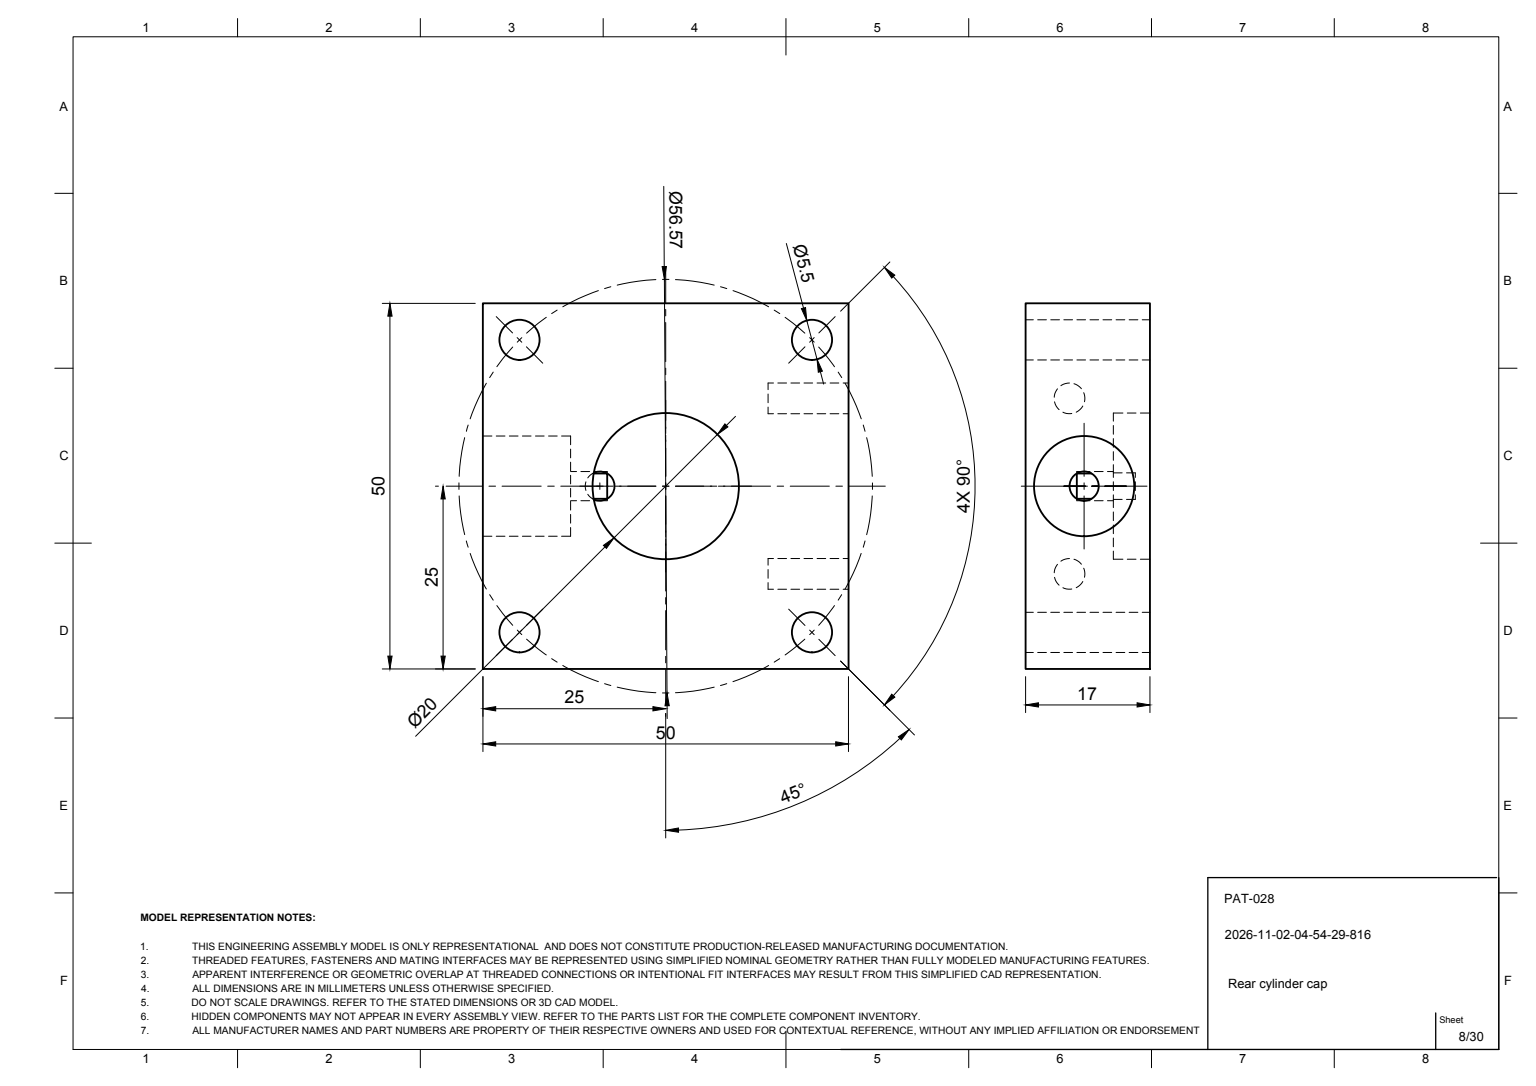
ISO-10303-21;
HEADER;
/* Generated by software containing ST-Developer
 * from STEP Tools, Inc. (www.steptools.com) 
 */

FILE_DESCRIPTION(
/* description */ ('Cylinder foot and clevis mount kit'),
/* implementation_level */ '2;1');

FILE_NAME(
/* name */ 'Rear cylinder cap.step',
/* time_stamp */ '2026-10-27T20:10:43-07:00',
/* author */ (''),
/* organization */ (''),
/* preprocessor_version */ 'ST-DEVELOPER v20.2',
/* originating_system */ 'Autodesk Translation Framework v15.17.0.0',
/* authorisation */ '');

FILE_SCHEMA (('AUTOMOTIVE_DESIGN { 1 0 10303 214 3 1 1 }'));
ENDSEC;

DATA;
#10=MECHANICAL_DESIGN_GEOMETRIC_PRESENTATION_REPRESENTATION('',(#341),#9102);
#285=SHAPE_REPRESENTATION_RELATIONSHIP('SRR','None',#9232,#313);
#313=ADVANCED_BREP_SHAPE_REPRESENTATION('',(#369),#9075);
#341=STYLED_ITEM('',(#9446),#369);
#369=MANIFOLD_SOLID_BREP('Body1',#4927);
#417=FACE_BOUND('',#1113,.T.);
#418=FACE_BOUND('',#1120,.T.);
#419=FACE_BOUND('',#1121,.T.);
#420=FACE_BOUND('',#1122,.T.);
#421=FACE_BOUND('',#1123,.T.);
#422=FACE_BOUND('',#1126,.T.);
#423=FACE_BOUND('',#1127,.T.);
#424=FACE_BOUND('',#1128,.T.);
#425=FACE_BOUND('',#1129,.T.);
#426=FACE_BOUND('',#1130,.T.);
#427=FACE_BOUND('',#1133,.T.);
#428=FACE_BOUND('',#1135,.T.);
#429=FACE_BOUND('',#1136,.T.);
#502=ELLIPSE('',#5409,0.282842712474618,0.2);
#503=ELLIPSE('',#5410,0.282842712474618,0.2);
#504=ELLIPSE('',#5411,0.282842712474618,0.2);
#505=ELLIPSE('',#5414,0.282842712474618,0.2);
#506=ELLIPSE('',#5415,0.282842712474618,0.2);
#507=ELLIPSE('',#5417,0.282842712474618,0.2);
#508=ELLIPSE('',#5418,0.282842712474618,0.2);
#550=PLANE('',#5395);
#551=PLANE('',#5399);
#552=PLANE('',#5400);
#553=PLANE('',#5402);
#554=PLANE('',#5404);
#555=PLANE('',#5419);
#556=PLANE('',#5421);
#557=PLANE('',#5423);
#558=PLANE('',#5425);
#559=PLANE('',#5431);
#560=PLANE('',#5437);
#561=PLANE('',#5452);
#562=PLANE('',#5453);
#563=PLANE('',#5454);
#564=PLANE('',#5455);
#565=PLANE('',#5456);
#566=PLANE('',#5457);
#762=FACE_OUTER_BOUND('',#1093,.T.);
#763=FACE_OUTER_BOUND('',#1094,.T.);
#764=FACE_OUTER_BOUND('',#1095,.T.);
#765=FACE_OUTER_BOUND('',#1096,.T.);
#766=FACE_OUTER_BOUND('',#1097,.T.);
#767=FACE_OUTER_BOUND('',#1098,.T.);
#768=FACE_OUTER_BOUND('',#1099,.T.);
#769=FACE_OUTER_BOUND('',#1100,.T.);
#770=FACE_OUTER_BOUND('',#1101,.T.);
#771=FACE_OUTER_BOUND('',#1102,.T.);
#772=FACE_OUTER_BOUND('',#1103,.T.);
#773=FACE_OUTER_BOUND('',#1104,.T.);
#774=FACE_OUTER_BOUND('',#1105,.T.);
#775=FACE_OUTER_BOUND('',#1106,.T.);
#776=FACE_OUTER_BOUND('',#1107,.T.);
#777=FACE_OUTER_BOUND('',#1108,.T.);
#778=FACE_OUTER_BOUND('',#1109,.T.);
#779=FACE_OUTER_BOUND('',#1110,.T.);
#780=FACE_OUTER_BOUND('',#1111,.T.);
#781=FACE_OUTER_BOUND('',#1112,.T.);
#782=FACE_OUTER_BOUND('',#1114,.T.);
#783=FACE_OUTER_BOUND('',#1115,.T.);
#784=FACE_OUTER_BOUND('',#1116,.T.);
#785=FACE_OUTER_BOUND('',#1117,.T.);
#786=FACE_OUTER_BOUND('',#1118,.T.);
#787=FACE_OUTER_BOUND('',#1119,.T.);
#788=FACE_OUTER_BOUND('',#1124,.T.);
#789=FACE_OUTER_BOUND('',#1125,.T.);
#790=FACE_OUTER_BOUND('',#1131,.T.);
#791=FACE_OUTER_BOUND('',#1132,.T.);
#792=FACE_OUTER_BOUND('',#1134,.T.);
#1093=EDGE_LOOP('',(#3591,#3592,#3593,#3594));
#1094=EDGE_LOOP('',(#3595));
#1095=EDGE_LOOP('',(#3596,#3597,#3598,#3599));
#1096=EDGE_LOOP('',(#3600));
#1097=EDGE_LOOP('',(#3601,#3602));
#1098=EDGE_LOOP('',(#3603,#3604));
#1099=EDGE_LOOP('',(#3605,#3606));
#1100=EDGE_LOOP('',(#3607,#3608,#3609,#3610,#3611,#3612,#3613,#3614,#3615,
#3616,#3617,#3618,#3619));
#1101=EDGE_LOOP('',(#3620,#3621,#3622));
#1102=EDGE_LOOP('',(#3623,#3624,#3625));
#1103=EDGE_LOOP('',(#3626,#3627));
#1104=EDGE_LOOP('',(#3628,#3629));
#1105=EDGE_LOOP('',(#3630,#3631));
#1106=EDGE_LOOP('',(#3632,#3633));
#1107=EDGE_LOOP('',(#3634,#3635,#3636));
#1108=EDGE_LOOP('',(#3637,#3638,#3639));
#1109=EDGE_LOOP('',(#3640,#3641,#3642,#3643,#3644,#3645,#3646,#3647,#3648));
#1110=EDGE_LOOP('',(#3649,#3650,#3651,#3652));
#1111=EDGE_LOOP('',(#3653,#3654,#3655,#3656));
#1112=EDGE_LOOP('',(#3657));
#1113=EDGE_LOOP('',(#3658));
#1114=EDGE_LOOP('',(#3659,#3660,#3661,#3662));
#1115=EDGE_LOOP('',(#3663,#3664,#3665,#3666));
#1116=EDGE_LOOP('',(#3667,#3668,#3669,#3670));
#1117=EDGE_LOOP('',(#3671,#3672,#3673,#3674));
#1118=EDGE_LOOP('',(#3675,#3676,#3677,#3678,#3679,#3680,#3681,#3682));
#1119=EDGE_LOOP('',(#3683,#3684,#3685,#3686));
#1120=EDGE_LOOP('',(#3687));
#1121=EDGE_LOOP('',(#3688));
#1122=EDGE_LOOP('',(#3689));
#1123=EDGE_LOOP('',(#3690));
#1124=EDGE_LOOP('',(#3691,#3692,#3693,#3694));
#1125=EDGE_LOOP('',(#3695,#3696,#3697,#3698));
#1126=EDGE_LOOP('',(#3699));
#1127=EDGE_LOOP('',(#3700));
#1128=EDGE_LOOP('',(#3701));
#1129=EDGE_LOOP('',(#3702));
#1130=EDGE_LOOP('',(#3703));
#1131=EDGE_LOOP('',(#3704,#3705,#3706,#3707));
#1132=EDGE_LOOP('',(#3708,#3709,#3710,#3711));
#1133=EDGE_LOOP('',(#3712));
#1134=EDGE_LOOP('',(#3713,#3714,#3715,#3716));
#1135=EDGE_LOOP('',(#3717));
#1136=EDGE_LOOP('',(#3718));
#1492=LINE('',#7797,#1841);
#1493=LINE('',#7804,#1842);
#1494=LINE('',#7810,#1843);
#1495=LINE('',#7814,#1844);
#1496=LINE('',#7818,#1845);
#1497=LINE('',#7823,#1846);
#1498=LINE('',#7827,#1847);
#1499=LINE('',#7831,#1848);
#1500=LINE('',#7836,#1849);
#1501=LINE('',#7838,#1850);
#1502=LINE('',#7859,#1851);
#1503=LINE('',#7869,#1852);
#1504=LINE('',#7876,#1853);
#1505=LINE('',#7882,#1854);
#1506=LINE('',#7888,#1855);
#1507=LINE('',#7894,#1856);
#1508=LINE('',#7899,#1857);
#1509=LINE('',#7903,#1858);
#1510=LINE('',#7905,#1859);
#1511=LINE('',#7907,#1860);
#1512=LINE('',#7908,#1861);
#1513=LINE('',#7911,#1862);
#1514=LINE('',#7913,#1863);
#1515=LINE('',#7914,#1864);
#1516=LINE('',#7917,#1865);
#1517=LINE('',#7919,#1866);
#1518=LINE('',#7920,#1867);
#1519=LINE('',#7922,#1868);
#1520=LINE('',#7923,#1869);
#1841=VECTOR('',#6235,0.21);
#1842=VECTOR('',#6244,0.21);
#1843=VECTOR('',#6251,1.);
#1844=VECTOR('',#6256,1.);
#1845=VECTOR('',#6261,1.);
#1846=VECTOR('',#6266,1.);
#1847=VECTOR('',#6269,1.);
#1848=VECTOR('',#6272,0.2);
#1849=VECTOR('',#6277,1.);
#1850=VECTOR('',#6278,1.);
#1851=VECTOR('',#6317,0.2);
#1852=VECTOR('',#6330,0.685);
#1853=VECTOR('',#6339,0.275);
#1854=VECTOR('',#6346,0.275);
#1855=VECTOR('',#6353,0.275);
#1856=VECTOR('',#6360,0.275);
#1857=VECTOR('',#6367,1.);
#1858=VECTOR('',#6370,1.);
#1859=VECTOR('',#6371,1.);
#1860=VECTOR('',#6372,1.);
#1861=VECTOR('',#6373,1.);
#1862=VECTOR('',#6376,1.);
#1863=VECTOR('',#6377,1.);
#1864=VECTOR('',#6378,1.);
#1865=VECTOR('',#6381,1.);
#1866=VECTOR('',#6382,1.);
#1867=VECTOR('',#6383,1.);
#1868=VECTOR('',#6386,1.);
#1869=VECTOR('',#6387,1.);
#2157=CIRCLE('',#5393,0.21);
#2158=CIRCLE('',#5394,0.21);
#2159=CIRCLE('',#5397,0.21);
#2160=CIRCLE('',#5398,0.21);
#2161=CIRCLE('',#5401,0.2);
#2162=CIRCLE('',#5403,0.2);
#2163=CIRCLE('',#5405,0.2);
#2164=CIRCLE('',#5407,0.2);
#2165=CIRCLE('',#5408,0.2);
#2166=CIRCLE('',#5412,0.2);
#2167=CIRCLE('',#5420,1.);
#2168=CIRCLE('',#5422,0.2);
#2169=CIRCLE('',#5424,0.2);
#2170=CIRCLE('',#5426,0.2);
#2171=CIRCLE('',#5430,0.2);
#2172=CIRCLE('',#5432,1.);
#2173=CIRCLE('',#5433,1.);
#2174=CIRCLE('',#5435,0.685);
#2175=CIRCLE('',#5436,0.685);
#2176=CIRCLE('',#5439,0.275);
#2177=CIRCLE('',#5440,0.275);
#2178=CIRCLE('',#5442,0.275);
#2179=CIRCLE('',#5443,0.275);
#2180=CIRCLE('',#5445,0.275);
#2181=CIRCLE('',#5446,0.275);
#2182=CIRCLE('',#5448,0.275);
#2183=CIRCLE('',#5449,0.275);
#2184=CIRCLE('',#5451,1.);
#2414=VERTEX_POINT('',#7794);
#2415=VERTEX_POINT('',#7796);
#2416=VERTEX_POINT('',#7801);
#2417=VERTEX_POINT('',#7803);
#2418=VERTEX_POINT('',#7808);
#2419=VERTEX_POINT('',#7809);
#2420=VERTEX_POINT('',#7813);
#2421=VERTEX_POINT('',#7817);
#2422=VERTEX_POINT('',#7821);
#2423=VERTEX_POINT('',#7822);
#2424=VERTEX_POINT('',#7824);
#2425=VERTEX_POINT('',#7826);
#2426=VERTEX_POINT('',#7828);
#2427=VERTEX_POINT('',#7830);
#2428=VERTEX_POINT('',#7832);
#2429=VERTEX_POINT('',#7834);
#2430=VERTEX_POINT('',#7837);
#2431=VERTEX_POINT('',#7858);
#2432=VERTEX_POINT('',#7862);
#2433=VERTEX_POINT('',#7866);
#2434=VERTEX_POINT('',#7868);
#2435=VERTEX_POINT('',#7873);
#2436=VERTEX_POINT('',#7875);
#2437=VERTEX_POINT('',#7879);
#2438=VERTEX_POINT('',#7881);
#2439=VERTEX_POINT('',#7885);
#2440=VERTEX_POINT('',#7887);
#2441=VERTEX_POINT('',#7891);
#2442=VERTEX_POINT('',#7893);
#2443=VERTEX_POINT('',#7897);
#2444=VERTEX_POINT('',#7901);
#2445=VERTEX_POINT('',#7902);
#2446=VERTEX_POINT('',#7904);
#2447=VERTEX_POINT('',#7906);
#2448=VERTEX_POINT('',#7910);
#2449=VERTEX_POINT('',#7912);
#2450=VERTEX_POINT('',#7916);
#2451=VERTEX_POINT('',#7918);
#2850=EDGE_CURVE('',#2414,#2414,#2157,.T.);
#2851=EDGE_CURVE('',#2414,#2415,#1492,.T.);
#2852=EDGE_CURVE('',#2415,#2415,#2158,.T.);
#2853=EDGE_CURVE('',#2416,#2416,#2159,.T.);
#2854=EDGE_CURVE('',#2416,#2417,#1493,.T.);
#2855=EDGE_CURVE('',#2417,#2417,#2160,.T.);
#2856=EDGE_CURVE('',#2418,#2419,#1494,.T.);
#2857=EDGE_CURVE('',#2419,#2418,#2161,.T.);
#2858=EDGE_CURVE('',#2419,#2420,#1495,.T.);
#2859=EDGE_CURVE('',#2420,#2419,#2162,.T.);
#2860=EDGE_CURVE('',#2421,#2418,#1496,.T.);
#2861=EDGE_CURVE('',#2418,#2421,#2163,.T.);
#2862=EDGE_CURVE('',#2422,#2423,#1497,.T.);
#2863=EDGE_CURVE('',#2424,#2422,#2164,.T.);
#2864=EDGE_CURVE('',#2425,#2424,#1498,.T.);
#2865=EDGE_CURVE('',#2426,#2425,#2165,.T.);
#2866=EDGE_CURVE('',#2426,#2427,#1499,.T.);
#2867=EDGE_CURVE('',#2428,#2427,#502,.T.);
#2868=EDGE_CURVE('',#2429,#2428,#503,.T.);
#2869=EDGE_CURVE('',#2419,#2429,#1500,.T.);
#2870=EDGE_CURVE('',#2430,#2418,#1501,.T.);
#2871=EDGE_CURVE('',#2427,#2430,#504,.T.);
#2872=EDGE_CURVE('',#2423,#2426,#2166,.T.);
#2873=EDGE_CURVE('',#2420,#2428,#505,.T.);
#2874=EDGE_CURVE('',#2428,#2419,#506,.T.);
#2875=EDGE_CURVE('',#2427,#2421,#507,.T.);
#2876=EDGE_CURVE('',#2418,#2427,#508,.T.);
#2877=EDGE_CURVE('',#2424,#2422,#2167,.T.);
#2878=EDGE_CURVE('',#2419,#2418,#2168,.T.);
#2879=EDGE_CURVE('',#2429,#2419,#2169,.T.);
#2880=EDGE_CURVE('',#2418,#2430,#2170,.T.);
#2881=EDGE_CURVE('',#2427,#2431,#1502,.T.);
#2882=EDGE_CURVE('',#2431,#2431,#2171,.T.);
#2883=EDGE_CURVE('',#2432,#2425,#2172,.T.);
#2884=EDGE_CURVE('',#2423,#2432,#2173,.T.);
#2885=EDGE_CURVE('',#2433,#2433,#2174,.T.);
#2886=EDGE_CURVE('',#2433,#2434,#1503,.T.);
#2887=EDGE_CURVE('',#2434,#2434,#2175,.T.);
#2888=EDGE_CURVE('',#2435,#2435,#2176,.T.);
#2889=EDGE_CURVE('',#2435,#2436,#1504,.T.);
#2890=EDGE_CURVE('',#2436,#2436,#2177,.T.);
#2891=EDGE_CURVE('',#2437,#2437,#2178,.T.);
#2892=EDGE_CURVE('',#2437,#2438,#1505,.T.);
#2893=EDGE_CURVE('',#2438,#2438,#2179,.T.);
#2894=EDGE_CURVE('',#2439,#2439,#2180,.T.);
#2895=EDGE_CURVE('',#2439,#2440,#1506,.T.);
#2896=EDGE_CURVE('',#2440,#2440,#2181,.T.);
#2897=EDGE_CURVE('',#2441,#2441,#2182,.T.);
#2898=EDGE_CURVE('',#2441,#2442,#1507,.T.);
#2899=EDGE_CURVE('',#2442,#2442,#2183,.T.);
#2900=EDGE_CURVE('',#2443,#2443,#2184,.T.);
#2901=EDGE_CURVE('',#2443,#2432,#1508,.T.);
#2902=EDGE_CURVE('',#2444,#2445,#1509,.T.);
#2903=EDGE_CURVE('',#2445,#2446,#1510,.T.);
#2904=EDGE_CURVE('',#2447,#2446,#1511,.T.);
#2905=EDGE_CURVE('',#2444,#2447,#1512,.T.);
#2906=EDGE_CURVE('',#2448,#2444,#1513,.T.);
#2907=EDGE_CURVE('',#2449,#2447,#1514,.T.);
#2908=EDGE_CURVE('',#2448,#2449,#1515,.T.);
#2909=EDGE_CURVE('',#2450,#2448,#1516,.T.);
#2910=EDGE_CURVE('',#2451,#2449,#1517,.T.);
#2911=EDGE_CURVE('',#2450,#2451,#1518,.T.);
#2912=EDGE_CURVE('',#2445,#2450,#1519,.T.);
#2913=EDGE_CURVE('',#2446,#2451,#1520,.T.);
#3591=ORIENTED_EDGE('',*,*,#2850,.F.);
#3592=ORIENTED_EDGE('',*,*,#2851,.T.);
#3593=ORIENTED_EDGE('',*,*,#2852,.T.);
#3594=ORIENTED_EDGE('',*,*,#2851,.F.);
#3595=ORIENTED_EDGE('',*,*,#2852,.F.);
#3596=ORIENTED_EDGE('',*,*,#2853,.F.);
#3597=ORIENTED_EDGE('',*,*,#2854,.T.);
#3598=ORIENTED_EDGE('',*,*,#2855,.T.);
#3599=ORIENTED_EDGE('',*,*,#2854,.F.);
#3600=ORIENTED_EDGE('',*,*,#2855,.F.);
#3601=ORIENTED_EDGE('',*,*,#2856,.F.);
#3602=ORIENTED_EDGE('',*,*,#2857,.F.);
#3603=ORIENTED_EDGE('',*,*,#2858,.F.);
#3604=ORIENTED_EDGE('',*,*,#2859,.F.);
#3605=ORIENTED_EDGE('',*,*,#2860,.F.);
#3606=ORIENTED_EDGE('',*,*,#2861,.F.);
#3607=ORIENTED_EDGE('',*,*,#2862,.F.);
#3608=ORIENTED_EDGE('',*,*,#2863,.F.);
#3609=ORIENTED_EDGE('',*,*,#2864,.F.);
#3610=ORIENTED_EDGE('',*,*,#2865,.F.);
#3611=ORIENTED_EDGE('',*,*,#2866,.T.);
#3612=ORIENTED_EDGE('',*,*,#2867,.F.);
#3613=ORIENTED_EDGE('',*,*,#2868,.F.);
#3614=ORIENTED_EDGE('',*,*,#2869,.F.);
#3615=ORIENTED_EDGE('',*,*,#2857,.T.);
#3616=ORIENTED_EDGE('',*,*,#2870,.F.);
#3617=ORIENTED_EDGE('',*,*,#2871,.F.);
#3618=ORIENTED_EDGE('',*,*,#2866,.F.);
#3619=ORIENTED_EDGE('',*,*,#2872,.F.);
#3620=ORIENTED_EDGE('',*,*,#2873,.F.);
#3621=ORIENTED_EDGE('',*,*,#2859,.T.);
#3622=ORIENTED_EDGE('',*,*,#2874,.F.);
#3623=ORIENTED_EDGE('',*,*,#2875,.F.);
#3624=ORIENTED_EDGE('',*,*,#2876,.F.);
#3625=ORIENTED_EDGE('',*,*,#2861,.T.);
#3626=ORIENTED_EDGE('',*,*,#2877,.F.);
#3627=ORIENTED_EDGE('',*,*,#2863,.T.);
#3628=ORIENTED_EDGE('',*,*,#2856,.T.);
#3629=ORIENTED_EDGE('',*,*,#2878,.T.);
#3630=ORIENTED_EDGE('',*,*,#2869,.T.);
#3631=ORIENTED_EDGE('',*,*,#2879,.T.);
#3632=ORIENTED_EDGE('',*,*,#2870,.T.);
#3633=ORIENTED_EDGE('',*,*,#2880,.T.);
#3634=ORIENTED_EDGE('',*,*,#2874,.T.);
#3635=ORIENTED_EDGE('',*,*,#2879,.F.);
#3636=ORIENTED_EDGE('',*,*,#2868,.T.);
#3637=ORIENTED_EDGE('',*,*,#2871,.T.);
#3638=ORIENTED_EDGE('',*,*,#2880,.F.);
#3639=ORIENTED_EDGE('',*,*,#2876,.T.);
#3640=ORIENTED_EDGE('',*,*,#2860,.T.);
#3641=ORIENTED_EDGE('',*,*,#2878,.F.);
#3642=ORIENTED_EDGE('',*,*,#2858,.T.);
#3643=ORIENTED_EDGE('',*,*,#2873,.T.);
#3644=ORIENTED_EDGE('',*,*,#2867,.T.);
#3645=ORIENTED_EDGE('',*,*,#2881,.T.);
#3646=ORIENTED_EDGE('',*,*,#2882,.F.);
#3647=ORIENTED_EDGE('',*,*,#2881,.F.);
#3648=ORIENTED_EDGE('',*,*,#2875,.T.);
#3649=ORIENTED_EDGE('',*,*,#2872,.T.);
#3650=ORIENTED_EDGE('',*,*,#2865,.T.);
#3651=ORIENTED_EDGE('',*,*,#2883,.F.);
#3652=ORIENTED_EDGE('',*,*,#2884,.F.);
#3653=ORIENTED_EDGE('',*,*,#2885,.F.);
#3654=ORIENTED_EDGE('',*,*,#2886,.T.);
#3655=ORIENTED_EDGE('',*,*,#2887,.F.);
#3656=ORIENTED_EDGE('',*,*,#2886,.F.);
#3657=ORIENTED_EDGE('',*,*,#2885,.T.);
#3658=ORIENTED_EDGE('',*,*,#2882,.T.);
#3659=ORIENTED_EDGE('',*,*,#2888,.F.);
#3660=ORIENTED_EDGE('',*,*,#2889,.T.);
#3661=ORIENTED_EDGE('',*,*,#2890,.F.);
#3662=ORIENTED_EDGE('',*,*,#2889,.F.);
#3663=ORIENTED_EDGE('',*,*,#2891,.F.);
#3664=ORIENTED_EDGE('',*,*,#2892,.T.);
#3665=ORIENTED_EDGE('',*,*,#2893,.F.);
#3666=ORIENTED_EDGE('',*,*,#2892,.F.);
#3667=ORIENTED_EDGE('',*,*,#2894,.F.);
#3668=ORIENTED_EDGE('',*,*,#2895,.T.);
#3669=ORIENTED_EDGE('',*,*,#2896,.F.);
#3670=ORIENTED_EDGE('',*,*,#2895,.F.);
#3671=ORIENTED_EDGE('',*,*,#2897,.F.);
#3672=ORIENTED_EDGE('',*,*,#2898,.T.);
#3673=ORIENTED_EDGE('',*,*,#2899,.F.);
#3674=ORIENTED_EDGE('',*,*,#2898,.F.);
#3675=ORIENTED_EDGE('',*,*,#2900,.F.);
#3676=ORIENTED_EDGE('',*,*,#2901,.T.);
#3677=ORIENTED_EDGE('',*,*,#2883,.T.);
#3678=ORIENTED_EDGE('',*,*,#2864,.T.);
#3679=ORIENTED_EDGE('',*,*,#2877,.T.);
#3680=ORIENTED_EDGE('',*,*,#2862,.T.);
#3681=ORIENTED_EDGE('',*,*,#2884,.T.);
#3682=ORIENTED_EDGE('',*,*,#2901,.F.);
#3683=ORIENTED_EDGE('',*,*,#2902,.T.);
#3684=ORIENTED_EDGE('',*,*,#2903,.T.);
#3685=ORIENTED_EDGE('',*,*,#2904,.F.);
#3686=ORIENTED_EDGE('',*,*,#2905,.F.);
#3687=ORIENTED_EDGE('',*,*,#2890,.T.);
#3688=ORIENTED_EDGE('',*,*,#2893,.T.);
#3689=ORIENTED_EDGE('',*,*,#2896,.T.);
#3690=ORIENTED_EDGE('',*,*,#2899,.T.);
#3691=ORIENTED_EDGE('',*,*,#2906,.T.);
#3692=ORIENTED_EDGE('',*,*,#2905,.T.);
#3693=ORIENTED_EDGE('',*,*,#2907,.F.);
#3694=ORIENTED_EDGE('',*,*,#2908,.F.);
#3695=ORIENTED_EDGE('',*,*,#2909,.T.);
#3696=ORIENTED_EDGE('',*,*,#2908,.T.);
#3697=ORIENTED_EDGE('',*,*,#2910,.F.);
#3698=ORIENTED_EDGE('',*,*,#2911,.F.);
#3699=ORIENTED_EDGE('',*,*,#2900,.T.);
#3700=ORIENTED_EDGE('',*,*,#2897,.T.);
#3701=ORIENTED_EDGE('',*,*,#2894,.T.);
#3702=ORIENTED_EDGE('',*,*,#2891,.T.);
#3703=ORIENTED_EDGE('',*,*,#2888,.T.);
#3704=ORIENTED_EDGE('',*,*,#2912,.T.);
#3705=ORIENTED_EDGE('',*,*,#2911,.T.);
#3706=ORIENTED_EDGE('',*,*,#2913,.F.);
#3707=ORIENTED_EDGE('',*,*,#2903,.F.);
#3708=ORIENTED_EDGE('',*,*,#2913,.T.);
#3709=ORIENTED_EDGE('',*,*,#2910,.T.);
#3710=ORIENTED_EDGE('',*,*,#2907,.T.);
#3711=ORIENTED_EDGE('',*,*,#2904,.T.);
#3712=ORIENTED_EDGE('',*,*,#2887,.T.);
#3713=ORIENTED_EDGE('',*,*,#2912,.F.);
#3714=ORIENTED_EDGE('',*,*,#2902,.F.);
#3715=ORIENTED_EDGE('',*,*,#2906,.F.);
#3716=ORIENTED_EDGE('',*,*,#2909,.F.);
#3717=ORIENTED_EDGE('',*,*,#2850,.T.);
#3718=ORIENTED_EDGE('',*,*,#2853,.T.);
#4545=CYLINDRICAL_SURFACE('',#5392,0.21);
#4546=CYLINDRICAL_SURFACE('',#5396,0.21);
#4547=CYLINDRICAL_SURFACE('',#5406,0.2);
#4548=CYLINDRICAL_SURFACE('',#5413,0.2);
#4549=CYLINDRICAL_SURFACE('',#5416,0.2);
#4550=CYLINDRICAL_SURFACE('',#5427,0.2);
#4551=CYLINDRICAL_SURFACE('',#5428,0.2);
#4552=CYLINDRICAL_SURFACE('',#5429,0.2);
#4553=CYLINDRICAL_SURFACE('',#5434,0.685);
#4554=CYLINDRICAL_SURFACE('',#5438,0.275);
#4555=CYLINDRICAL_SURFACE('',#5441,0.275);
#4556=CYLINDRICAL_SURFACE('',#5444,0.275);
#4557=CYLINDRICAL_SURFACE('',#5447,0.275);
#4558=CYLINDRICAL_SURFACE('',#5450,1.);
#4685=ADVANCED_FACE('',(#762),#4545,.F.);
#4686=ADVANCED_FACE('',(#763),#550,.F.);
#4687=ADVANCED_FACE('',(#764),#4546,.F.);
#4688=ADVANCED_FACE('',(#765),#551,.F.);
#4689=ADVANCED_FACE('',(#766),#552,.F.);
#4690=ADVANCED_FACE('',(#767),#553,.F.);
#4691=ADVANCED_FACE('',(#768),#554,.F.);
#4692=ADVANCED_FACE('',(#769),#4547,.F.);
#4693=ADVANCED_FACE('',(#770),#4548,.F.);
#4694=ADVANCED_FACE('',(#771),#4549,.F.);
#4695=ADVANCED_FACE('',(#772),#555,.T.);
#4696=ADVANCED_FACE('',(#773),#556,.T.);
#4697=ADVANCED_FACE('',(#774),#557,.T.);
#4698=ADVANCED_FACE('',(#775),#558,.T.);
#4699=ADVANCED_FACE('',(#776),#4550,.F.);
#4700=ADVANCED_FACE('',(#777),#4551,.F.);
#4701=ADVANCED_FACE('',(#778),#4552,.F.);
#4702=ADVANCED_FACE('',(#779),#559,.F.);
#4703=ADVANCED_FACE('',(#780),#4553,.F.);
#4704=ADVANCED_FACE('',(#781,#417),#560,.T.);
#4705=ADVANCED_FACE('',(#782),#4554,.F.);
#4706=ADVANCED_FACE('',(#783),#4555,.F.);
#4707=ADVANCED_FACE('',(#784),#4556,.F.);
#4708=ADVANCED_FACE('',(#785),#4557,.F.);
#4709=ADVANCED_FACE('',(#786),#4558,.F.);
#4710=ADVANCED_FACE('',(#787,#418,#419,#420,#421),#561,.T.);
#4711=ADVANCED_FACE('',(#788),#562,.T.);
#4712=ADVANCED_FACE('',(#789,#422,#423,#424,#425,#426),#563,.T.);
#4713=ADVANCED_FACE('',(#790),#564,.T.);
#4714=ADVANCED_FACE('',(#791,#427),#565,.T.);
#4715=ADVANCED_FACE('',(#792,#428,#429),#566,.F.);
#4927=CLOSED_SHELL('',(#4685,#4686,#4687,#4688,#4689,#4690,#4691,#4692,
#4693,#4694,#4695,#4696,#4697,#4698,#4699,#4700,#4701,#4702,#4703,#4704,
#4705,#4706,#4707,#4708,#4709,#4710,#4711,#4712,#4713,#4714,#4715));
#5391=AXIS2_PLACEMENT_3D('',#7792,#6229,#6230);
#5392=AXIS2_PLACEMENT_3D('',#7793,#6231,#6232);
#5393=AXIS2_PLACEMENT_3D('',#7795,#6233,#6234);
#5394=AXIS2_PLACEMENT_3D('',#7798,#6236,#6237);
#5395=AXIS2_PLACEMENT_3D('',#7799,#6238,#6239);
#5396=AXIS2_PLACEMENT_3D('',#7800,#6240,#6241);
#5397=AXIS2_PLACEMENT_3D('',#7802,#6242,#6243);
#5398=AXIS2_PLACEMENT_3D('',#7805,#6245,#6246);
#5399=AXIS2_PLACEMENT_3D('',#7806,#6247,#6248);
#5400=AXIS2_PLACEMENT_3D('',#7807,#6249,#6250);
#5401=AXIS2_PLACEMENT_3D('',#7811,#6252,#6253);
#5402=AXIS2_PLACEMENT_3D('',#7812,#6254,#6255);
#5403=AXIS2_PLACEMENT_3D('',#7815,#6257,#6258);
#5404=AXIS2_PLACEMENT_3D('',#7816,#6259,#6260);
#5405=AXIS2_PLACEMENT_3D('',#7819,#6262,#6263);
#5406=AXIS2_PLACEMENT_3D('',#7820,#6264,#6265);
#5407=AXIS2_PLACEMENT_3D('',#7825,#6267,#6268);
#5408=AXIS2_PLACEMENT_3D('',#7829,#6270,#6271);
#5409=AXIS2_PLACEMENT_3D('',#7833,#6273,#6274);
#5410=AXIS2_PLACEMENT_3D('',#7835,#6275,#6276);
#5411=AXIS2_PLACEMENT_3D('',#7839,#6279,#6280);
#5412=AXIS2_PLACEMENT_3D('',#7840,#6281,#6282);
#5413=AXIS2_PLACEMENT_3D('',#7841,#6283,#6284);
#5414=AXIS2_PLACEMENT_3D('',#7842,#6285,#6286);
#5415=AXIS2_PLACEMENT_3D('',#7843,#6287,#6288);
#5416=AXIS2_PLACEMENT_3D('',#7844,#6289,#6290);
#5417=AXIS2_PLACEMENT_3D('',#7845,#6291,#6292);
#5418=AXIS2_PLACEMENT_3D('',#7846,#6293,#6294);
#5419=AXIS2_PLACEMENT_3D('',#7847,#6295,#6296);
#5420=AXIS2_PLACEMENT_3D('',#7848,#6297,#6298);
#5421=AXIS2_PLACEMENT_3D('',#7849,#6299,#6300);
#5422=AXIS2_PLACEMENT_3D('',#7850,#6301,#6302);
#5423=AXIS2_PLACEMENT_3D('',#7851,#6303,#6304);
#5424=AXIS2_PLACEMENT_3D('',#7852,#6305,#6306);
#5425=AXIS2_PLACEMENT_3D('',#7853,#6307,#6308);
#5426=AXIS2_PLACEMENT_3D('',#7854,#6309,#6310);
#5427=AXIS2_PLACEMENT_3D('',#7855,#6311,#6312);
#5428=AXIS2_PLACEMENT_3D('',#7856,#6313,#6314);
#5429=AXIS2_PLACEMENT_3D('',#7857,#6315,#6316);
#5430=AXIS2_PLACEMENT_3D('',#7860,#6318,#6319);
#5431=AXIS2_PLACEMENT_3D('',#7861,#6320,#6321);
#5432=AXIS2_PLACEMENT_3D('',#7863,#6322,#6323);
#5433=AXIS2_PLACEMENT_3D('',#7864,#6324,#6325);
#5434=AXIS2_PLACEMENT_3D('',#7865,#6326,#6327);
#5435=AXIS2_PLACEMENT_3D('',#7867,#6328,#6329);
#5436=AXIS2_PLACEMENT_3D('',#7870,#6331,#6332);
#5437=AXIS2_PLACEMENT_3D('',#7871,#6333,#6334);
#5438=AXIS2_PLACEMENT_3D('',#7872,#6335,#6336);
#5439=AXIS2_PLACEMENT_3D('',#7874,#6337,#6338);
#5440=AXIS2_PLACEMENT_3D('',#7877,#6340,#6341);
#5441=AXIS2_PLACEMENT_3D('',#7878,#6342,#6343);
#5442=AXIS2_PLACEMENT_3D('',#7880,#6344,#6345);
#5443=AXIS2_PLACEMENT_3D('',#7883,#6347,#6348);
#5444=AXIS2_PLACEMENT_3D('',#7884,#6349,#6350);
#5445=AXIS2_PLACEMENT_3D('',#7886,#6351,#6352);
#5446=AXIS2_PLACEMENT_3D('',#7889,#6354,#6355);
#5447=AXIS2_PLACEMENT_3D('',#7890,#6356,#6357);
#5448=AXIS2_PLACEMENT_3D('',#7892,#6358,#6359);
#5449=AXIS2_PLACEMENT_3D('',#7895,#6361,#6362);
#5450=AXIS2_PLACEMENT_3D('',#7896,#6363,#6364);
#5451=AXIS2_PLACEMENT_3D('',#7898,#6365,#6366);
#5452=AXIS2_PLACEMENT_3D('',#7900,#6368,#6369);
#5453=AXIS2_PLACEMENT_3D('',#7909,#6374,#6375);
#5454=AXIS2_PLACEMENT_3D('',#7915,#6379,#6380);
#5455=AXIS2_PLACEMENT_3D('',#7921,#6384,#6385);
#5456=AXIS2_PLACEMENT_3D('',#7924,#6388,#6389);
#5457=AXIS2_PLACEMENT_3D('',#7925,#6390,#6391);
#6229=DIRECTION('axis',(0.,0.,1.));
#6230=DIRECTION('refdir',(1.,0.,0.));
#6231=DIRECTION('center_axis',(0.,0.,1.));
#6232=DIRECTION('ref_axis',(1.,0.,0.));
#6233=DIRECTION('center_axis',(0.,0.,1.));
#6234=DIRECTION('ref_axis',(1.,0.,0.));
#6235=DIRECTION('',(0.,0.,1.));
#6236=DIRECTION('center_axis',(0.,0.,1.));
#6237=DIRECTION('ref_axis',(1.,0.,0.));
#6238=DIRECTION('center_axis',(0.,0.,1.));
#6239=DIRECTION('ref_axis',(1.,0.,0.));
#6240=DIRECTION('center_axis',(0.,0.,1.));
#6241=DIRECTION('ref_axis',(1.,0.,0.));
#6242=DIRECTION('center_axis',(0.,0.,1.));
#6243=DIRECTION('ref_axis',(1.,0.,0.));
#6244=DIRECTION('',(0.,0.,1.));
#6245=DIRECTION('center_axis',(0.,0.,1.));
#6246=DIRECTION('ref_axis',(1.,0.,0.));
#6247=DIRECTION('center_axis',(0.,0.,1.));
#6248=DIRECTION('ref_axis',(1.,0.,0.));
#6249=DIRECTION('center_axis',(0.,1.,0.));
#6250=DIRECTION('ref_axis',(1.,0.,0.));
#6251=DIRECTION('',(1.,0.,0.));
#6252=DIRECTION('center_axis',(0.,1.,0.));
#6253=DIRECTION('ref_axis',(1.,0.,0.));
#6254=DIRECTION('center_axis',(0.,1.,0.));
#6255=DIRECTION('ref_axis',(1.,0.,0.));
#6256=DIRECTION('',(0.,0.,1.));
#6257=DIRECTION('center_axis',(0.,1.,0.));
#6258=DIRECTION('ref_axis',(1.,0.,0.));
#6259=DIRECTION('center_axis',(0.,1.,0.));
#6260=DIRECTION('ref_axis',(1.,0.,0.));
#6261=DIRECTION('',(0.,0.,-1.));
#6262=DIRECTION('center_axis',(0.,1.,0.));
#6263=DIRECTION('ref_axis',(1.,0.,0.));
#6264=DIRECTION('center_axis',(0.,1.,0.));
#6265=DIRECTION('ref_axis',(1.,0.,0.));
#6266=DIRECTION('',(0.,1.,0.));
#6267=DIRECTION('center_axis',(0.,1.,0.));
#6268=DIRECTION('ref_axis',(1.,0.,0.));
#6269=DIRECTION('',(0.,-1.,0.));
#6270=DIRECTION('center_axis',(0.,1.,0.));
#6271=DIRECTION('ref_axis',(1.,0.,0.));
#6272=DIRECTION('',(0.,1.,0.));
#6273=DIRECTION('center_axis',(0.,-0.707106781186549,-0.707106781186546));
#6274=DIRECTION('ref_axis',(0.,0.707106781186546,-0.707106781186549));
#6275=DIRECTION('center_axis',(0.,-0.707106781186549,0.707106781186546));
#6276=DIRECTION('ref_axis',(0.,-0.707106781186546,-0.707106781186549));
#6277=DIRECTION('',(0.,-1.,0.));
#6278=DIRECTION('',(0.,1.,0.));
#6279=DIRECTION('center_axis',(0.,-0.707106781186549,0.707106781186546));
#6280=DIRECTION('ref_axis',(0.,-0.707106781186546,-0.707106781186549));
#6281=DIRECTION('center_axis',(0.,1.,0.));
#6282=DIRECTION('ref_axis',(1.,0.,0.));
#6283=DIRECTION('center_axis',(0.,1.,0.));
#6284=DIRECTION('ref_axis',(1.,0.,0.));
#6285=DIRECTION('center_axis',(0.,0.707106781186549,-0.707106781186546));
#6286=DIRECTION('ref_axis',(0.,-0.707106781186546,-0.707106781186549));
#6287=DIRECTION('center_axis',(0.,0.707106781186549,0.707106781186546));
#6288=DIRECTION('ref_axis',(0.,0.707106781186546,-0.707106781186549));
#6289=DIRECTION('center_axis',(0.,1.,0.));
#6290=DIRECTION('ref_axis',(-1.,0.,1.22464679914735E-16));
#6291=DIRECTION('center_axis',(0.,0.707106781186549,-0.707106781186546));
#6292=DIRECTION('ref_axis',(0.,-0.707106781186546,-0.707106781186549));
#6293=DIRECTION('center_axis',(0.,0.707106781186549,0.707106781186546));
#6294=DIRECTION('ref_axis',(0.,0.707106781186546,-0.707106781186549));
#6295=DIRECTION('center_axis',(0.,1.,0.));
#6296=DIRECTION('ref_axis',(1.,0.,0.));
#6297=DIRECTION('center_axis',(0.,1.,0.));
#6298=DIRECTION('ref_axis',(1.,0.,0.));
#6299=DIRECTION('center_axis',(0.,0.,1.));
#6300=DIRECTION('ref_axis',(1.,0.,0.));
#6301=DIRECTION('center_axis',(0.,0.,1.));
#6302=DIRECTION('ref_axis',(1.,0.,0.));
#6303=DIRECTION('center_axis',(0.,0.,1.));
#6304=DIRECTION('ref_axis',(1.,0.,0.));
#6305=DIRECTION('center_axis',(0.,0.,1.));
#6306=DIRECTION('ref_axis',(1.,0.,0.));
#6307=DIRECTION('center_axis',(0.,0.,1.));
#6308=DIRECTION('ref_axis',(1.,0.,0.));
#6309=DIRECTION('center_axis',(0.,0.,1.));
#6310=DIRECTION('ref_axis',(1.,0.,0.));
#6311=DIRECTION('center_axis',(0.,0.,1.));
#6312=DIRECTION('ref_axis',(1.,0.,0.));
#6313=DIRECTION('center_axis',(0.,0.,1.));
#6314=DIRECTION('ref_axis',(-1.,5.20660583828602E-15,0.));
#6315=DIRECTION('center_axis',(0.,0.,1.));
#6316=DIRECTION('ref_axis',(1.,0.,0.));
#6317=DIRECTION('',(0.,0.,1.));
#6318=DIRECTION('center_axis',(0.,0.,-1.));
#6319=DIRECTION('ref_axis',(1.,0.,0.));
#6320=DIRECTION('center_axis',(0.,1.,0.));
#6321=DIRECTION('ref_axis',(1.,0.,0.));
#6322=DIRECTION('center_axis',(0.,1.,0.));
#6323=DIRECTION('ref_axis',(1.,0.,0.));
#6324=DIRECTION('center_axis',(0.,1.,0.));
#6325=DIRECTION('ref_axis',(1.,0.,0.));
#6326=DIRECTION('center_axis',(0.,0.,1.));
#6327=DIRECTION('ref_axis',(1.,0.,0.));
#6328=DIRECTION('center_axis',(0.,0.,1.));
#6329=DIRECTION('ref_axis',(1.,0.,0.));
#6330=DIRECTION('',(0.,0.,1.));
#6331=DIRECTION('center_axis',(0.,0.,-1.));
#6332=DIRECTION('ref_axis',(1.,0.,0.));
#6333=DIRECTION('center_axis',(0.,0.,1.));
#6334=DIRECTION('ref_axis',(1.,0.,0.));
#6335=DIRECTION('center_axis',(0.,1.,0.));
#6336=DIRECTION('ref_axis',(1.,0.,0.));
#6337=DIRECTION('center_axis',(0.,1.,0.));
#6338=DIRECTION('ref_axis',(1.,0.,0.));
#6339=DIRECTION('',(0.,1.,0.));
#6340=DIRECTION('center_axis',(0.,-1.,0.));
#6341=DIRECTION('ref_axis',(1.,0.,0.));
#6342=DIRECTION('center_axis',(0.,1.,0.));
#6343=DIRECTION('ref_axis',(1.,0.,0.));
#6344=DIRECTION('center_axis',(0.,1.,0.));
#6345=DIRECTION('ref_axis',(1.,0.,0.));
#6346=DIRECTION('',(0.,1.,0.));
#6347=DIRECTION('center_axis',(0.,-1.,0.));
#6348=DIRECTION('ref_axis',(1.,0.,0.));
#6349=DIRECTION('center_axis',(0.,1.,0.));
#6350=DIRECTION('ref_axis',(1.,0.,0.));
#6351=DIRECTION('center_axis',(0.,1.,0.));
#6352=DIRECTION('ref_axis',(1.,0.,0.));
#6353=DIRECTION('',(0.,1.,0.));
#6354=DIRECTION('center_axis',(0.,-1.,0.));
#6355=DIRECTION('ref_axis',(1.,0.,0.));
#6356=DIRECTION('center_axis',(0.,1.,0.));
#6357=DIRECTION('ref_axis',(1.,0.,0.));
#6358=DIRECTION('center_axis',(0.,1.,0.));
#6359=DIRECTION('ref_axis',(1.,0.,0.));
#6360=DIRECTION('',(0.,1.,0.));
#6361=DIRECTION('center_axis',(0.,-1.,0.));
#6362=DIRECTION('ref_axis',(1.,0.,0.));
#6363=DIRECTION('center_axis',(0.,1.,0.));
#6364=DIRECTION('ref_axis',(1.,0.,0.));
#6365=DIRECTION('center_axis',(0.,1.,0.));
#6366=DIRECTION('ref_axis',(1.,0.,0.));
#6367=DIRECTION('',(0.,1.,0.));
#6368=DIRECTION('center_axis',(0.,1.,0.));
#6369=DIRECTION('ref_axis',(-1.,0.,0.));
#6370=DIRECTION('',(-1.,0.,0.));
#6371=DIRECTION('',(0.,0.,1.));
#6372=DIRECTION('',(-1.,0.,0.));
#6373=DIRECTION('',(0.,0.,1.));
#6374=DIRECTION('center_axis',(1.,0.,0.));
#6375=DIRECTION('ref_axis',(0.,1.,0.));
#6376=DIRECTION('',(0.,1.,0.));
#6377=DIRECTION('',(0.,1.,0.));
#6378=DIRECTION('',(0.,0.,1.));
#6379=DIRECTION('center_axis',(0.,-1.,0.));
#6380=DIRECTION('ref_axis',(1.,0.,0.));
#6381=DIRECTION('',(1.,0.,0.));
#6382=DIRECTION('',(1.,0.,0.));
#6383=DIRECTION('',(0.,0.,1.));
#6384=DIRECTION('center_axis',(-1.,0.,0.));
#6385=DIRECTION('ref_axis',(0.,-1.,0.));
#6386=DIRECTION('',(0.,-1.,0.));
#6387=DIRECTION('',(0.,-1.,0.));
#6388=DIRECTION('center_axis',(0.,0.,1.));
#6389=DIRECTION('ref_axis',(1.,0.,0.));
#6390=DIRECTION('center_axis',(0.,0.,1.));
#6391=DIRECTION('ref_axis',(1.,0.,0.));
#7792=CARTESIAN_POINT('',(0.,0.,0.));
#7793=CARTESIAN_POINT('Origin',(-1.2,12.,1.9));
#7794=CARTESIAN_POINT('',(-1.41,12.,2.));
#7795=CARTESIAN_POINT('Origin',(-1.2,12.,2.));
#7796=CARTESIAN_POINT('',(-1.41,12.,3.1));
#7797=CARTESIAN_POINT('',(-1.41,12.,1.9));
#7798=CARTESIAN_POINT('Origin',(-1.2,12.,3.1));
#7799=CARTESIAN_POINT('Origin',(-1.2,12.,3.1));
#7800=CARTESIAN_POINT('Origin',(1.2,12.,1.9));
#7801=CARTESIAN_POINT('',(0.99,12.,2.));
#7802=CARTESIAN_POINT('Origin',(1.2,12.,2.));
#7803=CARTESIAN_POINT('',(0.99,12.,3.1));
#7804=CARTESIAN_POINT('',(0.99,12.,1.9));
#7805=CARTESIAN_POINT('Origin',(1.2,12.,3.1));
#7806=CARTESIAN_POINT('Origin',(1.2,12.,3.1));
#7807=CARTESIAN_POINT('Origin',(0.,11.9,5.4));
#7808=CARTESIAN_POINT('',(-0.173205080756887,11.9,5.3));
#7809=CARTESIAN_POINT('',(0.173205080756887,11.9,5.3));
#7810=CARTESIAN_POINT('',(0.,11.9,5.3));
#7811=CARTESIAN_POINT('Origin',(0.,11.9,5.4));
#7812=CARTESIAN_POINT('Origin',(0.,11.9,5.4));
#7813=CARTESIAN_POINT('',(0.173205080756887,11.9,5.5));
#7814=CARTESIAN_POINT('',(0.173205080756887,11.9,5.3));
#7815=CARTESIAN_POINT('Origin',(0.,11.9,5.4));
#7816=CARTESIAN_POINT('Origin',(0.,11.9,5.4));
#7817=CARTESIAN_POINT('',(-0.173205080756887,11.9,5.5));
#7818=CARTESIAN_POINT('',(-0.173205080756887,11.9,5.3));
#7819=CARTESIAN_POINT('Origin',(0.,11.9,5.4));
#7820=CARTESIAN_POINT('Origin',(0.,11.1,5.4));
#7821=CARTESIAN_POINT('',(0.181811868577262,11.1,5.48333333333333));
#7822=CARTESIAN_POINT('',(0.181811868577262,11.4,5.48333333333333));
#7823=CARTESIAN_POINT('',(0.181811868577262,11.1,5.48333333333333));
#7824=CARTESIAN_POINT('',(-0.181811868577262,11.1,5.48333333333333));
#7825=CARTESIAN_POINT('Origin',(0.,11.1,5.4));
#7826=CARTESIAN_POINT('',(-0.181811868577262,11.4,5.48333333333333));
#7827=CARTESIAN_POINT('',(-0.181811868577262,11.1,5.48333333333333));
#7828=CARTESIAN_POINT('',(-0.2,11.4,5.4));
#7829=CARTESIAN_POINT('Origin',(0.,11.4,5.4));
#7830=CARTESIAN_POINT('',(-0.2,11.8,5.4));
#7831=CARTESIAN_POINT('',(-0.2,11.1,5.4));
#7832=CARTESIAN_POINT('',(0.2,11.8,5.4));
#7833=CARTESIAN_POINT('Origin',(0.,11.8,5.4));
#7834=CARTESIAN_POINT('',(0.173205080756888,11.7,5.3));
#7835=CARTESIAN_POINT('Origin',(0.,11.8,5.4));
#7836=CARTESIAN_POINT('',(0.173205080756888,11.1,5.3));
#7837=CARTESIAN_POINT('',(-0.173205080756888,11.7,5.3));
#7838=CARTESIAN_POINT('',(-0.173205080756888,11.1,5.3));
#7839=CARTESIAN_POINT('Origin',(0.,11.8,5.4));
#7840=CARTESIAN_POINT('Origin',(0.,11.4,5.4));
#7841=CARTESIAN_POINT('Origin',(0.,11.1,5.4));
#7842=CARTESIAN_POINT('Origin',(0.,11.8,5.4));
#7843=CARTESIAN_POINT('Origin',(0.,11.8,5.4));
#7844=CARTESIAN_POINT('Origin',(0.,11.1,5.4));
#7845=CARTESIAN_POINT('Origin',(0.,11.8,5.4));
#7846=CARTESIAN_POINT('Origin',(0.,11.8,5.4));
#7847=CARTESIAN_POINT('Origin',(0.,11.1,5.4));
#7848=CARTESIAN_POINT('Origin',(0.,11.1,4.5));
#7849=CARTESIAN_POINT('Origin',(0.,11.8,5.3));
#7850=CARTESIAN_POINT('Origin',(0.,11.8,5.3));
#7851=CARTESIAN_POINT('Origin',(0.,11.8,5.3));
#7852=CARTESIAN_POINT('Origin',(0.,11.8,5.3));
#7853=CARTESIAN_POINT('Origin',(0.,11.8,5.3));
#7854=CARTESIAN_POINT('Origin',(0.,11.8,5.3));
#7855=CARTESIAN_POINT('Origin',(0.,11.8,5.3));
#7856=CARTESIAN_POINT('Origin',(0.,11.8,5.3));
#7857=CARTESIAN_POINT('Origin',(0.,11.8,5.3));
#7858=CARTESIAN_POINT('',(-0.2,11.8,5.8));
#7859=CARTESIAN_POINT('',(-0.2,11.8,5.3));
#7860=CARTESIAN_POINT('Origin',(0.,11.8,5.8));
#7861=CARTESIAN_POINT('Origin',(0.,11.4,4.5));
#7862=CARTESIAN_POINT('',(-1.,11.4,4.5));
#7863=CARTESIAN_POINT('Origin',(0.,11.4,4.5));
#7864=CARTESIAN_POINT('Origin',(0.,11.4,4.5));
#7865=CARTESIAN_POINT('Origin',(0.,11.8,5.8));
#7866=CARTESIAN_POINT('',(-0.685,11.8,5.8));
#7867=CARTESIAN_POINT('Origin',(0.,11.8,5.8));
#7868=CARTESIAN_POINT('',(-0.685,11.8,7.));
#7869=CARTESIAN_POINT('',(-0.685,11.8,5.8));
#7870=CARTESIAN_POINT('Origin',(0.,11.8,7.));
#7871=CARTESIAN_POINT('Origin',(0.,11.8,5.8));
#7872=CARTESIAN_POINT('Origin',(2.,10.8,2.5));
#7873=CARTESIAN_POINT('',(1.725,10.9,2.5));
#7874=CARTESIAN_POINT('Origin',(2.,10.9,2.5));
#7875=CARTESIAN_POINT('',(1.725,12.6,2.5));
#7876=CARTESIAN_POINT('',(1.725,10.8,2.5));
#7877=CARTESIAN_POINT('Origin',(2.,12.6,2.5));
#7878=CARTESIAN_POINT('Origin',(-2.,10.8,6.5));
#7879=CARTESIAN_POINT('',(-2.275,10.9,6.5));
#7880=CARTESIAN_POINT('Origin',(-2.,10.9,6.5));
#7881=CARTESIAN_POINT('',(-2.275,12.6,6.5));
#7882=CARTESIAN_POINT('',(-2.275,10.8,6.5));
#7883=CARTESIAN_POINT('Origin',(-2.,12.6,6.5));
#7884=CARTESIAN_POINT('Origin',(-2.,10.8,2.5));
#7885=CARTESIAN_POINT('',(-2.275,10.9,2.5));
#7886=CARTESIAN_POINT('Origin',(-2.,10.9,2.5));
#7887=CARTESIAN_POINT('',(-2.275,12.6,2.5));
#7888=CARTESIAN_POINT('',(-2.275,10.8,2.5));
#7889=CARTESIAN_POINT('Origin',(-2.,12.6,2.5));
#7890=CARTESIAN_POINT('Origin',(2.,10.8,6.5));
#7891=CARTESIAN_POINT('',(1.725,10.9,6.5));
#7892=CARTESIAN_POINT('Origin',(2.,10.9,6.5));
#7893=CARTESIAN_POINT('',(1.725,12.6,6.5));
#7894=CARTESIAN_POINT('',(1.725,10.8,6.5));
#7895=CARTESIAN_POINT('Origin',(2.,12.6,6.5));
#7896=CARTESIAN_POINT('Origin',(0.,10.8,4.5));
#7897=CARTESIAN_POINT('',(-1.,10.9,4.5));
#7898=CARTESIAN_POINT('Origin',(0.,10.9,4.5));
#7899=CARTESIAN_POINT('',(-1.,10.8,4.5));
#7900=CARTESIAN_POINT('Origin',(2.5,12.6,2.));
#7901=CARTESIAN_POINT('',(2.5,12.6,2.));
#7902=CARTESIAN_POINT('',(-2.5,12.6,2.));
#7903=CARTESIAN_POINT('',(2.5,12.6,2.));
#7904=CARTESIAN_POINT('',(-2.5,12.6,7.));
#7905=CARTESIAN_POINT('',(-2.5,12.6,2.));
#7906=CARTESIAN_POINT('',(2.5,12.6,7.));
#7907=CARTESIAN_POINT('',(2.5,12.6,7.));
#7908=CARTESIAN_POINT('',(2.5,12.6,2.));
#7909=CARTESIAN_POINT('Origin',(2.5,10.9,2.));
#7910=CARTESIAN_POINT('',(2.5,10.9,2.));
#7911=CARTESIAN_POINT('',(2.5,10.9,2.));
#7912=CARTESIAN_POINT('',(2.5,10.9,7.));
#7913=CARTESIAN_POINT('',(2.5,10.9,7.));
#7914=CARTESIAN_POINT('',(2.5,10.9,2.));
#7915=CARTESIAN_POINT('Origin',(-2.5,10.9,2.));
#7916=CARTESIAN_POINT('',(-2.5,10.9,2.));
#7917=CARTESIAN_POINT('',(-2.5,10.9,2.));
#7918=CARTESIAN_POINT('',(-2.5,10.9,7.));
#7919=CARTESIAN_POINT('',(-2.5,10.9,7.));
#7920=CARTESIAN_POINT('',(-2.5,10.9,2.));
#7921=CARTESIAN_POINT('Origin',(-2.5,12.6,2.));
#7922=CARTESIAN_POINT('',(-2.5,12.6,2.));
#7923=CARTESIAN_POINT('',(-2.5,12.6,7.));
#7924=CARTESIAN_POINT('Origin',(0.,11.75,7.));
#7925=CARTESIAN_POINT('Origin',(0.,11.75,2.));
#9042=UNCERTAINTY_MEASURE_WITH_UNIT(LENGTH_MEASURE(0.001),#9103,
'DISTANCE_ACCURACY_VALUE',
'Maximum model space distance between geometric entities at asserted c
onnectivities');
#9069=UNCERTAINTY_MEASURE_WITH_UNIT(LENGTH_MEASURE(0.001),#9103,
'DISTANCE_ACCURACY_VALUE',
'Maximum model space distance between geometric entities at asserted c
onnectivities');
#9075=(
GEOMETRIC_REPRESENTATION_CONTEXT(3)
GLOBAL_UNCERTAINTY_ASSIGNED_CONTEXT((#9042))
GLOBAL_UNIT_ASSIGNED_CONTEXT((#9103,#9105,#9106))
REPRESENTATION_CONTEXT('','3D')
);
#9102=(
GEOMETRIC_REPRESENTATION_CONTEXT(3)
GLOBAL_UNCERTAINTY_ASSIGNED_CONTEXT((#9069))
GLOBAL_UNIT_ASSIGNED_CONTEXT((#9103,#9105,#9106))
REPRESENTATION_CONTEXT('','3D')
);
#9103=(
LENGTH_UNIT()
NAMED_UNIT(*)
SI_UNIT(.CENTI.,.METRE.)
);
#9105=(
NAMED_UNIT(*)
PLANE_ANGLE_UNIT()
SI_UNIT($,.RADIAN.)
);
#9106=(
NAMED_UNIT(*)
SI_UNIT($,.STERADIAN.)
SOLID_ANGLE_UNIT()
);
#9112=SHAPE_DEFINITION_REPRESENTATION(#9144,#9232);
#9144=PRODUCT_DEFINITION_SHAPE('',$,#9265);
#9232=SHAPE_REPRESENTATION('',(#5391),#9075);
#9259=PRODUCT_DEFINITION_CONTEXT('part definition',#9357,'design');
#9265=PRODUCT_DEFINITION('Rear cylinder cap','Rear cylinder cap',#9297,
#9259);
#9297=PRODUCT_DEFINITION_FORMATION('',$,#9364);
#9357=APPLICATION_CONTEXT(
'Core Data for Automotive Mechanical Design Process');
#9358=PRODUCT_CONTEXT('part definition',#9357,'mechanical');
#9364=PRODUCT('Rear cylinder cap','Rear cylinder cap',
'Rear cylinder cap',(#9358));
#9440=COLOUR_RGB('Light Blue',0.38,0.62,0.78);
#9441=FILL_AREA_STYLE_COLOUR('',#9440);
#9442=FILL_AREA_STYLE('',(#9441));
#9443=SURFACE_STYLE_FILL_AREA(#9442);
#9444=SURFACE_SIDE_STYLE('',(#9443));
#9445=SURFACE_STYLE_USAGE(.BOTH.,#9444);
#9446=PRESENTATION_STYLE_ASSIGNMENT((#9445));
ENDSEC;
END-ISO-10303-21;
